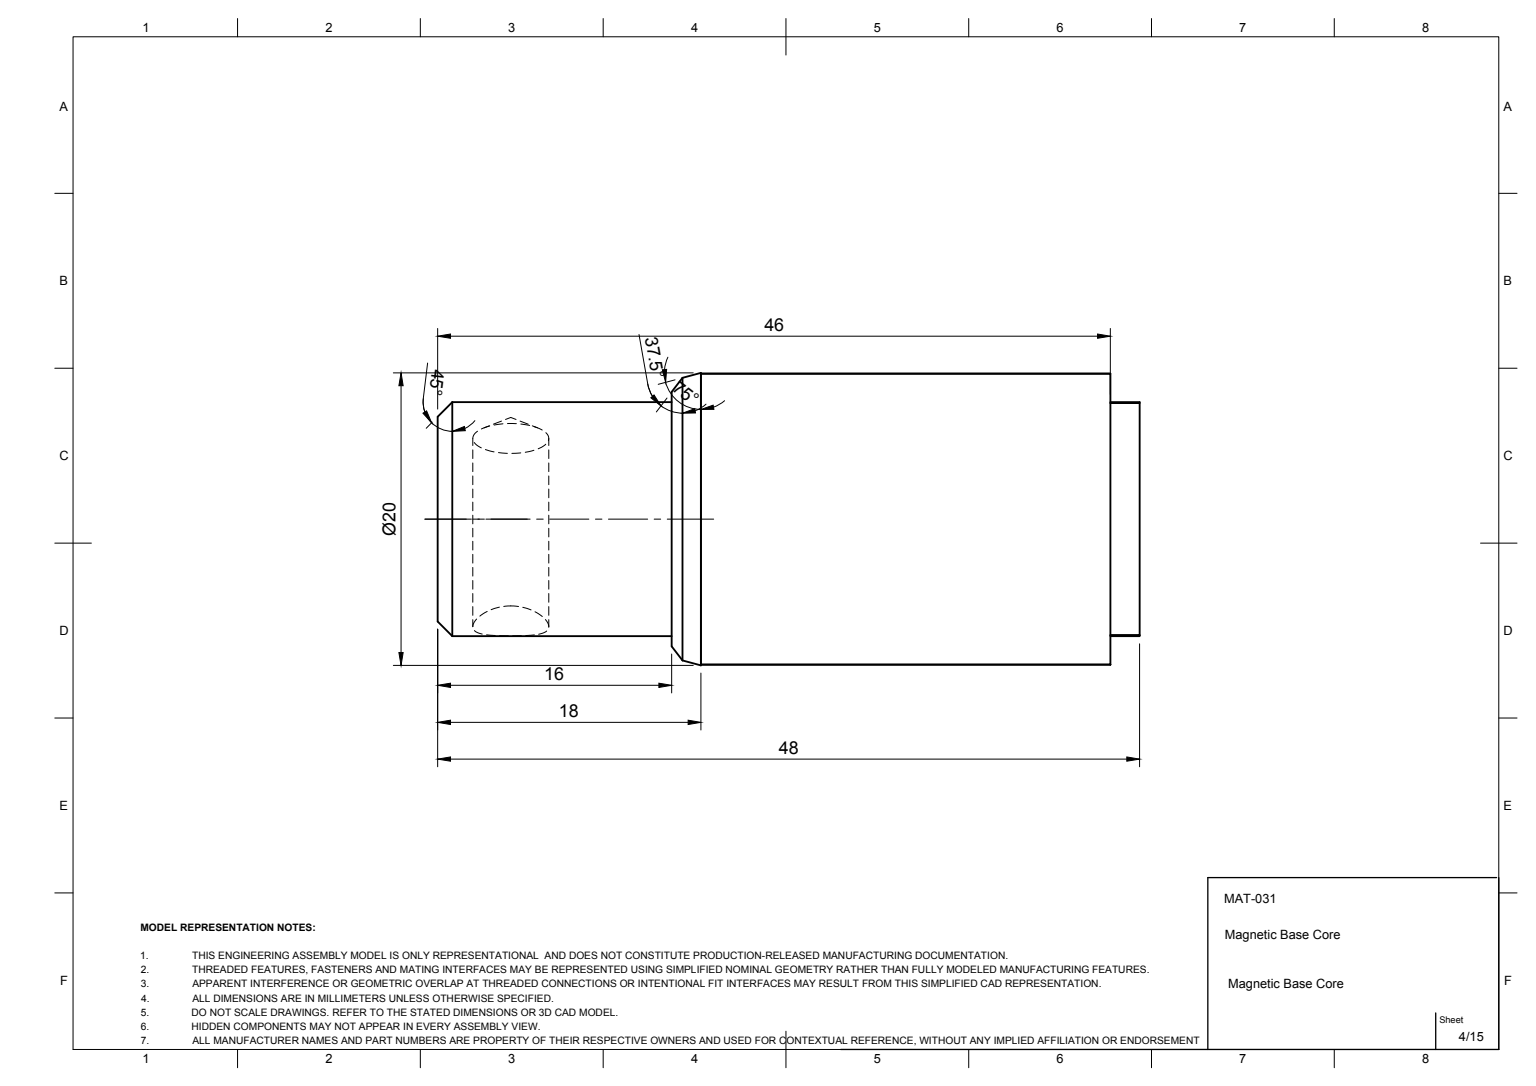
ISO-10303-21;
HEADER;
/* Generated by software containing ST-Developer
 * from STEP Tools, Inc. (www.steptools.com) 
 */

FILE_DESCRIPTION(
/* description */ ('STEP AP214'),
/* implementation_level */ '2;1');

FILE_NAME(
/* name */ 'Magnetic Base Core.step',
/* time_stamp */ '2026-11-14T06:58:01-08:00',
/* author */ (''),
/* organization */ (''),
/* preprocessor_version */ 'ST-DEVELOPER v20.2',
/* originating_system */ 'Autodesk Translation Framework v15.17.0.0',
/* authorisation */ '');

FILE_SCHEMA (('AUTOMOTIVE_DESIGN { 1 0 10303 214 3 1 1 }'));
ENDSEC;

DATA;
#10=MECHANICAL_DESIGN_GEOMETRIC_PRESENTATION_REPRESENTATION('',(#1144,#1145,#1146,#1147),#38635);
#862=FACE_BOUND('',#2714,.T.);
#863=FACE_BOUND('',#2717,.T.);
#907=B_SPLINE_CURVE_WITH_KNOTS('',3,(#24912,#24913,#24914,#24915,#24916,
#24917,#24918,#24919,#24920,#24921,#24922,#24923,#24924,#24925,#24926,#24927,
#24928,#24929,#24930,#24931,#24932,#24933,#24934,#24935,#24936,#24937,#24938,
#24939,#24940,#24941,#24942,#24943,#24944,#24945),.UNSPECIFIED.,.T.,.F.,
(4,2,2,2,2,2,2,2,2,2,2,2,2,2,2,2,4),(-1.57949026336004,-1.48075154424537,
-1.38201282513069,-1.28331526132536,-1.18461769752003,-1.08592013371471,
-0.98722256990938,-0.888483850794701,-0.789745131680022,-0.691006412565344,
-0.592267693450665,-0.493570129645338,-0.394872565840011,-0.296175002034684,
-0.197477438229357,-0.0987387191146787,0.),.UNSPECIFIED.);
#1018=CONICAL_SURFACE('',#17892,2.6,1.02974425867665);
#1019=CONICAL_SURFACE('',#17895,7.,0.785398163397448);
#1020=CONICAL_SURFACE('',#17898,8.69677462715879,0.916297857297022);
#1021=CONICAL_SURFACE('',#17904,10.,0.261799387799149);
#1113=SHAPE_REPRESENTATION_RELATIONSHIP('SRR','None',#38686,#1127);
#1127=ADVANCED_BREP_SHAPE_REPRESENTATION('',(#1170,#1171,#1172,#1173),#38622);
#1144=STYLED_ITEM('',(#38765),#1170);
#1145=STYLED_ITEM('',(#38765),#1171);
#1146=STYLED_ITEM('',(#38765),#1172);
#1147=STYLED_ITEM('',(#38765),#1173);
#1170=MANIFOLD_SOLID_BREP('Body1',#17610);
#1171=MANIFOLD_SOLID_BREP('Body2',#17611);
#1172=MANIFOLD_SOLID_BREP('Body3',#17612);
#1173=MANIFOLD_SOLID_BREP('Body4',#17613);
#1218=PLANE('',#17861);
#1219=PLANE('',#17863);
#1220=PLANE('',#17864);
#1221=PLANE('',#17865);
#1222=PLANE('',#17874);
#1223=PLANE('',#17875);
#1224=PLANE('',#17876);
#1225=PLANE('',#17877);
#1226=PLANE('',#17878);
#1227=PLANE('',#17879);
#1228=PLANE('',#17880);
#1229=PLANE('',#17881);
#1230=PLANE('',#17882);
#1231=PLANE('',#17885);
#1232=PLANE('',#17888);
#1233=PLANE('',#17889);
#1234=PLANE('',#17906);
#1235=PLANE('',#17907);
#1236=PLANE('',#17908);
#1681=FACE_OUTER_BOUND('',#2687,.T.);
#1682=FACE_OUTER_BOUND('',#2688,.T.);
#1683=FACE_OUTER_BOUND('',#2689,.T.);
#1684=FACE_OUTER_BOUND('',#2690,.T.);
#1685=FACE_OUTER_BOUND('',#2691,.T.);
#1686=FACE_OUTER_BOUND('',#2692,.T.);
#1687=FACE_OUTER_BOUND('',#2693,.T.);
#1688=FACE_OUTER_BOUND('',#2694,.T.);
#1689=FACE_OUTER_BOUND('',#2695,.T.);
#1690=FACE_OUTER_BOUND('',#2696,.T.);
#1691=FACE_OUTER_BOUND('',#2697,.T.);
#1692=FACE_OUTER_BOUND('',#2698,.T.);
#1693=FACE_OUTER_BOUND('',#2699,.T.);
#1694=FACE_OUTER_BOUND('',#2700,.T.);
#1695=FACE_OUTER_BOUND('',#2701,.T.);
#1696=FACE_OUTER_BOUND('',#2702,.T.);
#1697=FACE_OUTER_BOUND('',#2703,.T.);
#1698=FACE_OUTER_BOUND('',#2704,.T.);
#1699=FACE_OUTER_BOUND('',#2705,.T.);
#1700=FACE_OUTER_BOUND('',#2706,.T.);
#1701=FACE_OUTER_BOUND('',#2707,.T.);
#1702=FACE_OUTER_BOUND('',#2708,.T.);
#1703=FACE_OUTER_BOUND('',#2709,.T.);
#1704=FACE_OUTER_BOUND('',#2710,.T.);
#1705=FACE_OUTER_BOUND('',#2711,.T.);
#1706=FACE_OUTER_BOUND('',#2712,.T.);
#1707=FACE_OUTER_BOUND('',#2713,.T.);
#1708=FACE_OUTER_BOUND('',#2715,.T.);
#1709=FACE_OUTER_BOUND('',#2716,.T.);
#1710=FACE_OUTER_BOUND('',#2718,.T.);
#1711=FACE_OUTER_BOUND('',#2719,.T.);
#2687=EDGE_LOOP('',(#11101,#11102,#11103,#11104));
#2688=EDGE_LOOP('',(#11105,#11106));
#2689=EDGE_LOOP('',(#11107,#11108,#11109,#11110,#11111,#11112,#11113,#11114));
#2690=EDGE_LOOP('',(#11115,#11116));
#2691=EDGE_LOOP('',(#11117,#11118,#11119,#11120));
#2692=EDGE_LOOP('',(#11121,#11122,#11123,#11124));
#2693=EDGE_LOOP('',(#11125,#11126,#11127,#11128));
#2694=EDGE_LOOP('',(#11129,#11130,#11131,#11132));
#2695=EDGE_LOOP('',(#11133,#11134));
#2696=EDGE_LOOP('',(#11135,#11136,#11137,#11138,#11139,#11140,#11141,#11142));
#2697=EDGE_LOOP('',(#11143,#11144));
#2698=EDGE_LOOP('',(#11145,#11146,#11147,#11148));
#2699=EDGE_LOOP('',(#11149,#11150,#11151,#11152));
#2700=EDGE_LOOP('',(#11153,#11154,#11155,#11156,#11157,#11158,#11159,#11160));
#2701=EDGE_LOOP('',(#11161,#11162,#11163,#11164));
#2702=EDGE_LOOP('',(#11165,#11166,#11167,#11168,#11169,#11170,#11171,#11172));
#2703=EDGE_LOOP('',(#11173,#11174,#11175,#11176));
#2704=EDGE_LOOP('',(#11177,#11178,#11179,#11180));
#2705=EDGE_LOOP('',(#11181,#11182,#11183,#11184));
#2706=EDGE_LOOP('',(#11185,#11186,#11187,#11188));
#2707=EDGE_LOOP('',(#11189,#11190,#11191,#11192));
#2708=EDGE_LOOP('',(#11193,#11194,#11195,#11196));
#2709=EDGE_LOOP('',(#11197,#11198,#11199));
#2710=EDGE_LOOP('',(#11200,#11201,#11202,#11203));
#2711=EDGE_LOOP('',(#11204,#11205,#11206,#11207));
#2712=EDGE_LOOP('',(#11208,#11209,#11210,#11211,#11212));
#2713=EDGE_LOOP('',(#11213,#11214,#11215,#11216));
#2714=EDGE_LOOP('',(#11217));
#2715=EDGE_LOOP('',(#11218,#11219,#11220,#11221,#11222));
#2716=EDGE_LOOP('',(#11223));
#2717=EDGE_LOOP('',(#11224));
#2718=EDGE_LOOP('',(#11225));
#2719=EDGE_LOOP('',(#11226));
#3766=LINE('',#24807,#4710);
#3767=LINE('',#24810,#4711);
#3768=LINE('',#24815,#4712);
#3769=LINE('',#24818,#4713);
#3770=LINE('',#24819,#4714);
#3771=LINE('',#24821,#4715);
#3772=LINE('',#24822,#4716);
#3773=LINE('',#24823,#4717);
#3774=LINE('',#24833,#4718);
#3775=LINE('',#24836,#4719);
#3776=LINE('',#24842,#4720);
#3777=LINE('',#24845,#4721);
#3778=LINE('',#24847,#4722);
#3779=LINE('',#24849,#4723);
#3780=LINE('',#24850,#4724);
#3781=LINE('',#24851,#4725);
#3782=LINE('',#24857,#4726);
#3783=LINE('',#24859,#4727);
#3784=LINE('',#24861,#4728);
#3785=LINE('',#24862,#4729);
#3786=LINE('',#24866,#4730);
#3787=LINE('',#24868,#4731);
#3788=LINE('',#24870,#4732);
#3789=LINE('',#24872,#4733);
#3790=LINE('',#24874,#4734);
#3791=LINE('',#24875,#4735);
#3792=LINE('',#24876,#4736);
#3793=LINE('',#24880,#4737);
#3794=LINE('',#24881,#4738);
#3795=LINE('',#24882,#4739);
#3796=LINE('',#24885,#4740);
#3797=LINE('',#24887,#4741);
#3798=LINE('',#24889,#4742);
#3799=LINE('',#24891,#4743);
#3800=LINE('',#24892,#4744);
#3801=LINE('',#24893,#4745);
#3802=LINE('',#24907,#4746);
#3803=LINE('',#24911,#4747);
#3804=LINE('',#24950,#4748);
#3805=LINE('',#24958,#4749);
#3806=LINE('',#24963,#4750);
#3807=LINE('',#24967,#4751);
#4710=VECTOR('',#19957,1000.);
#4711=VECTOR('',#19960,1000.);
#4712=VECTOR('',#19965,1000.);
#4713=VECTOR('',#19968,1000.);
#4714=VECTOR('',#19969,1000.);
#4715=VECTOR('',#19970,1000.);
#4716=VECTOR('',#19971,1000.);
#4717=VECTOR('',#19972,1000.);
#4718=VECTOR('',#19985,1000.);
#4719=VECTOR('',#19988,1000.);
#4720=VECTOR('',#19993,1000.);
#4721=VECTOR('',#19996,1000.);
#4722=VECTOR('',#19999,1000.);
#4723=VECTOR('',#20002,1000.);
#4724=VECTOR('',#20003,1000.);
#4725=VECTOR('',#20004,1000.);
#4726=VECTOR('',#20011,1000.);
#4727=VECTOR('',#20012,1000.);
#4728=VECTOR('',#20013,1000.);
#4729=VECTOR('',#20014,1000.);
#4730=VECTOR('',#20017,1000.);
#4731=VECTOR('',#20018,1000.);
#4732=VECTOR('',#20019,1000.);
#4733=VECTOR('',#20020,1000.);
#4734=VECTOR('',#20021,1000.);
#4735=VECTOR('',#20022,1000.);
#4736=VECTOR('',#20023,1000.);
#4737=VECTOR('',#20026,1000.);
#4738=VECTOR('',#20027,1000.);
#4739=VECTOR('',#20028,1000.);
#4740=VECTOR('',#20031,1000.);
#4741=VECTOR('',#20032,1000.);
#4742=VECTOR('',#20033,1000.);
#4743=VECTOR('',#20034,1000.);
#4744=VECTOR('',#20035,1000.);
#4745=VECTOR('',#20036,1000.);
#4746=VECTOR('',#20059,2.6);
#4747=VECTOR('',#20064,2.6);
#4748=VECTOR('',#20069,7.);
#4749=VECTOR('',#20078,8.69677462715879);
#4750=VECTOR('',#20085,8.);
#4751=VECTOR('',#20090,10.);
#5614=CIRCLE('',#17859,10.);
#5615=CIRCLE('',#17860,10.);
#5616=CIRCLE('',#17862,8.);
#5617=CIRCLE('',#17866,8.);
#5618=CIRCLE('',#17869,8.);
#5619=CIRCLE('',#17870,8.);
#5620=CIRCLE('',#17872,10.);
#5621=CIRCLE('',#17873,10.);
#5622=CIRCLE('',#17883,8.);
#5623=CIRCLE('',#17884,8.);
#5624=CIRCLE('',#17887,8.);
#5625=CIRCLE('',#17890,8.);
#5626=CIRCLE('',#17893,2.6);
#5627=CIRCLE('',#17896,8.);
#5628=CIRCLE('',#17897,7.);
#5629=CIRCLE('',#17899,9.66270045344786);
#5630=CIRCLE('',#17900,9.66270045344786);
#5631=CIRCLE('',#17901,8.69677462715879);
#5632=CIRCLE('',#17903,8.);
#5633=CIRCLE('',#17905,10.);
#6576=VERTEX_POINT('',#24803);
#6577=VERTEX_POINT('',#24804);
#6578=VERTEX_POINT('',#24806);
#6579=VERTEX_POINT('',#24808);
#6580=VERTEX_POINT('',#24812);
#6581=VERTEX_POINT('',#24813);
#6582=VERTEX_POINT('',#24817);
#6583=VERTEX_POINT('',#24820);
#6584=VERTEX_POINT('',#24829);
#6585=VERTEX_POINT('',#24830);
#6586=VERTEX_POINT('',#24832);
#6587=VERTEX_POINT('',#24834);
#6588=VERTEX_POINT('',#24838);
#6589=VERTEX_POINT('',#24839);
#6590=VERTEX_POINT('',#24841);
#6591=VERTEX_POINT('',#24843);
#6592=VERTEX_POINT('',#24855);
#6593=VERTEX_POINT('',#24856);
#6594=VERTEX_POINT('',#24858);
#6595=VERTEX_POINT('',#24860);
#6596=VERTEX_POINT('',#24864);
#6597=VERTEX_POINT('',#24865);
#6598=VERTEX_POINT('',#24867);
#6599=VERTEX_POINT('',#24869);
#6600=VERTEX_POINT('',#24871);
#6601=VERTEX_POINT('',#24873);
#6602=VERTEX_POINT('',#24878);
#6603=VERTEX_POINT('',#24879);
#6604=VERTEX_POINT('',#24884);
#6605=VERTEX_POINT('',#24886);
#6606=VERTEX_POINT('',#24888);
#6607=VERTEX_POINT('',#24890);
#6608=VERTEX_POINT('',#24905);
#6609=VERTEX_POINT('',#24906);
#6610=VERTEX_POINT('',#24910);
#6611=VERTEX_POINT('',#24947);
#6612=VERTEX_POINT('',#24949);
#6613=VERTEX_POINT('',#24953);
#6614=VERTEX_POINT('',#24954);
#6615=VERTEX_POINT('',#24957);
#6616=VERTEX_POINT('',#24961);
#6617=VERTEX_POINT('',#24965);
#8337=EDGE_CURVE('',#6576,#6577,#5614,.T.);
#8338=EDGE_CURVE('',#6576,#6578,#3766,.T.);
#8339=EDGE_CURVE('',#6579,#6578,#5615,.T.);
#8340=EDGE_CURVE('',#6579,#6577,#3767,.T.);
#8341=EDGE_CURVE('',#6580,#6581,#5616,.T.);
#8342=EDGE_CURVE('',#6581,#6580,#3768,.T.);
#8343=EDGE_CURVE('',#6577,#6582,#3769,.T.);
#8344=EDGE_CURVE('',#6579,#6578,#3770,.T.);
#8345=EDGE_CURVE('',#6583,#6576,#3771,.T.);
#8346=EDGE_CURVE('',#6580,#6583,#3772,.T.);
#8347=EDGE_CURVE('',#6582,#6581,#3773,.T.);
#8348=EDGE_CURVE('',#6583,#6582,#5617,.T.);
#8349=EDGE_CURVE('',#6584,#6585,#5618,.T.);
#8350=EDGE_CURVE('',#6585,#6586,#3774,.T.);
#8351=EDGE_CURVE('',#6587,#6586,#5619,.T.);
#8352=EDGE_CURVE('',#6587,#6584,#3775,.T.);
#8353=EDGE_CURVE('',#6588,#6589,#5620,.T.);
#8354=EDGE_CURVE('',#6588,#6590,#3776,.T.);
#8355=EDGE_CURVE('',#6591,#6590,#5621,.T.);
#8356=EDGE_CURVE('',#6591,#6589,#3777,.T.);
#8357=EDGE_CURVE('',#6586,#6587,#3778,.T.);
#8358=EDGE_CURVE('',#6590,#6585,#3779,.T.);
#8359=EDGE_CURVE('',#6588,#6589,#3780,.T.);
#8360=EDGE_CURVE('',#6584,#6591,#3781,.T.);
#8361=EDGE_CURVE('',#6592,#6593,#3782,.T.);
#8362=EDGE_CURVE('',#6592,#6594,#3783,.T.);
#8363=EDGE_CURVE('',#6594,#6595,#3784,.T.);
#8364=EDGE_CURVE('',#6593,#6595,#3785,.T.);
#8365=EDGE_CURVE('',#6596,#6597,#3786,.T.);
#8366=EDGE_CURVE('',#6596,#6598,#3787,.T.);
#8367=EDGE_CURVE('',#6598,#6599,#3788,.T.);
#8368=EDGE_CURVE('',#6599,#6600,#3789,.T.);
#8369=EDGE_CURVE('',#6600,#6601,#3790,.T.);
#8370=EDGE_CURVE('',#6601,#6592,#3791,.T.);
#8371=EDGE_CURVE('',#6597,#6593,#3792,.T.);
#8372=EDGE_CURVE('',#6602,#6603,#3793,.T.);
#8373=EDGE_CURVE('',#6602,#6596,#3794,.T.);
#8374=EDGE_CURVE('',#6603,#6597,#3795,.T.);
#8375=EDGE_CURVE('',#6594,#6604,#3796,.T.);
#8376=EDGE_CURVE('',#6604,#6605,#3797,.T.);
#8377=EDGE_CURVE('',#6605,#6606,#3798,.T.);
#8378=EDGE_CURVE('',#6606,#6607,#3799,.T.);
#8379=EDGE_CURVE('',#6607,#6602,#3800,.T.);
#8380=EDGE_CURVE('',#6595,#6603,#3801,.T.);
#8381=EDGE_CURVE('',#6605,#6600,#5622,.T.);
#8382=EDGE_CURVE('',#6599,#6606,#5623,.T.);
#8383=EDGE_CURVE('',#6598,#6607,#5624,.T.);
#8384=EDGE_CURVE('',#6604,#6601,#5625,.T.);
#8385=EDGE_CURVE('',#6608,#6609,#3802,.T.);
#8386=EDGE_CURVE('',#6609,#6609,#5626,.T.);
#8387=EDGE_CURVE('',#6609,#6610,#3803,.T.);
#8388=EDGE_CURVE('',#6610,#6610,#907,.T.);
#8389=EDGE_CURVE('',#6611,#6611,#5627,.T.);
#8390=EDGE_CURVE('',#6611,#6612,#3804,.T.);
#8391=EDGE_CURVE('',#6612,#6612,#5628,.T.);
#8392=EDGE_CURVE('',#6613,#6614,#5629,.T.);
#8393=EDGE_CURVE('',#6614,#6613,#5630,.T.);
#8394=EDGE_CURVE('',#6614,#6615,#3805,.T.);
#8395=EDGE_CURVE('',#6615,#6615,#5631,.T.);
#8396=EDGE_CURVE('',#6616,#6616,#5632,.T.);
#8397=EDGE_CURVE('',#6616,#6611,#3806,.T.);
#8398=EDGE_CURVE('',#6617,#6617,#5633,.T.);
#8399=EDGE_CURVE('',#6617,#6613,#3807,.T.);
#11101=ORIENTED_EDGE('',*,*,#8337,.F.);
#11102=ORIENTED_EDGE('',*,*,#8338,.T.);
#11103=ORIENTED_EDGE('',*,*,#8339,.F.);
#11104=ORIENTED_EDGE('',*,*,#8340,.T.);
#11105=ORIENTED_EDGE('',*,*,#8341,.T.);
#11106=ORIENTED_EDGE('',*,*,#8342,.T.);
#11107=ORIENTED_EDGE('',*,*,#8343,.F.);
#11108=ORIENTED_EDGE('',*,*,#8340,.F.);
#11109=ORIENTED_EDGE('',*,*,#8344,.T.);
#11110=ORIENTED_EDGE('',*,*,#8338,.F.);
#11111=ORIENTED_EDGE('',*,*,#8345,.F.);
#11112=ORIENTED_EDGE('',*,*,#8346,.F.);
#11113=ORIENTED_EDGE('',*,*,#8342,.F.);
#11114=ORIENTED_EDGE('',*,*,#8347,.F.);
#11115=ORIENTED_EDGE('',*,*,#8344,.F.);
#11116=ORIENTED_EDGE('',*,*,#8339,.T.);
#11117=ORIENTED_EDGE('',*,*,#8343,.T.);
#11118=ORIENTED_EDGE('',*,*,#8348,.F.);
#11119=ORIENTED_EDGE('',*,*,#8345,.T.);
#11120=ORIENTED_EDGE('',*,*,#8337,.T.);
#11121=ORIENTED_EDGE('',*,*,#8347,.T.);
#11122=ORIENTED_EDGE('',*,*,#8341,.F.);
#11123=ORIENTED_EDGE('',*,*,#8346,.T.);
#11124=ORIENTED_EDGE('',*,*,#8348,.T.);
#11125=ORIENTED_EDGE('',*,*,#8349,.T.);
#11126=ORIENTED_EDGE('',*,*,#8350,.T.);
#11127=ORIENTED_EDGE('',*,*,#8351,.F.);
#11128=ORIENTED_EDGE('',*,*,#8352,.T.);
#11129=ORIENTED_EDGE('',*,*,#8353,.F.);
#11130=ORIENTED_EDGE('',*,*,#8354,.T.);
#11131=ORIENTED_EDGE('',*,*,#8355,.F.);
#11132=ORIENTED_EDGE('',*,*,#8356,.T.);
#11133=ORIENTED_EDGE('',*,*,#8351,.T.);
#11134=ORIENTED_EDGE('',*,*,#8357,.T.);
#11135=ORIENTED_EDGE('',*,*,#8358,.F.);
#11136=ORIENTED_EDGE('',*,*,#8354,.F.);
#11137=ORIENTED_EDGE('',*,*,#8359,.T.);
#11138=ORIENTED_EDGE('',*,*,#8356,.F.);
#11139=ORIENTED_EDGE('',*,*,#8360,.F.);
#11140=ORIENTED_EDGE('',*,*,#8352,.F.);
#11141=ORIENTED_EDGE('',*,*,#8357,.F.);
#11142=ORIENTED_EDGE('',*,*,#8350,.F.);
#11143=ORIENTED_EDGE('',*,*,#8359,.F.);
#11144=ORIENTED_EDGE('',*,*,#8353,.T.);
#11145=ORIENTED_EDGE('',*,*,#8358,.T.);
#11146=ORIENTED_EDGE('',*,*,#8349,.F.);
#11147=ORIENTED_EDGE('',*,*,#8360,.T.);
#11148=ORIENTED_EDGE('',*,*,#8355,.T.);
#11149=ORIENTED_EDGE('',*,*,#8361,.F.);
#11150=ORIENTED_EDGE('',*,*,#8362,.T.);
#11151=ORIENTED_EDGE('',*,*,#8363,.T.);
#11152=ORIENTED_EDGE('',*,*,#8364,.F.);
#11153=ORIENTED_EDGE('',*,*,#8365,.F.);
#11154=ORIENTED_EDGE('',*,*,#8366,.T.);
#11155=ORIENTED_EDGE('',*,*,#8367,.T.);
#11156=ORIENTED_EDGE('',*,*,#8368,.T.);
#11157=ORIENTED_EDGE('',*,*,#8369,.T.);
#11158=ORIENTED_EDGE('',*,*,#8370,.T.);
#11159=ORIENTED_EDGE('',*,*,#8361,.T.);
#11160=ORIENTED_EDGE('',*,*,#8371,.F.);
#11161=ORIENTED_EDGE('',*,*,#8372,.F.);
#11162=ORIENTED_EDGE('',*,*,#8373,.T.);
#11163=ORIENTED_EDGE('',*,*,#8365,.T.);
#11164=ORIENTED_EDGE('',*,*,#8374,.F.);
#11165=ORIENTED_EDGE('',*,*,#8363,.F.);
#11166=ORIENTED_EDGE('',*,*,#8375,.T.);
#11167=ORIENTED_EDGE('',*,*,#8376,.T.);
#11168=ORIENTED_EDGE('',*,*,#8377,.T.);
#11169=ORIENTED_EDGE('',*,*,#8378,.T.);
#11170=ORIENTED_EDGE('',*,*,#8379,.T.);
#11171=ORIENTED_EDGE('',*,*,#8372,.T.);
#11172=ORIENTED_EDGE('',*,*,#8380,.F.);
#11173=ORIENTED_EDGE('',*,*,#8377,.F.);
#11174=ORIENTED_EDGE('',*,*,#8381,.T.);
#11175=ORIENTED_EDGE('',*,*,#8368,.F.);
#11176=ORIENTED_EDGE('',*,*,#8382,.T.);
#11177=ORIENTED_EDGE('',*,*,#8364,.T.);
#11178=ORIENTED_EDGE('',*,*,#8380,.T.);
#11179=ORIENTED_EDGE('',*,*,#8374,.T.);
#11180=ORIENTED_EDGE('',*,*,#8371,.T.);
#11181=ORIENTED_EDGE('',*,*,#8383,.T.);
#11182=ORIENTED_EDGE('',*,*,#8378,.F.);
#11183=ORIENTED_EDGE('',*,*,#8382,.F.);
#11184=ORIENTED_EDGE('',*,*,#8367,.F.);
#11185=ORIENTED_EDGE('',*,*,#8373,.F.);
#11186=ORIENTED_EDGE('',*,*,#8379,.F.);
#11187=ORIENTED_EDGE('',*,*,#8383,.F.);
#11188=ORIENTED_EDGE('',*,*,#8366,.F.);
#11189=ORIENTED_EDGE('',*,*,#8384,.F.);
#11190=ORIENTED_EDGE('',*,*,#8375,.F.);
#11191=ORIENTED_EDGE('',*,*,#8362,.F.);
#11192=ORIENTED_EDGE('',*,*,#8370,.F.);
#11193=ORIENTED_EDGE('',*,*,#8381,.F.);
#11194=ORIENTED_EDGE('',*,*,#8376,.F.);
#11195=ORIENTED_EDGE('',*,*,#8384,.T.);
#11196=ORIENTED_EDGE('',*,*,#8369,.F.);
#11197=ORIENTED_EDGE('',*,*,#8385,.T.);
#11198=ORIENTED_EDGE('',*,*,#8386,.T.);
#11199=ORIENTED_EDGE('',*,*,#8385,.F.);
#11200=ORIENTED_EDGE('',*,*,#8386,.F.);
#11201=ORIENTED_EDGE('',*,*,#8387,.T.);
#11202=ORIENTED_EDGE('',*,*,#8388,.F.);
#11203=ORIENTED_EDGE('',*,*,#8387,.F.);
#11204=ORIENTED_EDGE('',*,*,#8389,.F.);
#11205=ORIENTED_EDGE('',*,*,#8390,.T.);
#11206=ORIENTED_EDGE('',*,*,#8391,.F.);
#11207=ORIENTED_EDGE('',*,*,#8390,.F.);
#11208=ORIENTED_EDGE('',*,*,#8392,.F.);
#11209=ORIENTED_EDGE('',*,*,#8393,.F.);
#11210=ORIENTED_EDGE('',*,*,#8394,.T.);
#11211=ORIENTED_EDGE('',*,*,#8395,.F.);
#11212=ORIENTED_EDGE('',*,*,#8394,.F.);
#11213=ORIENTED_EDGE('',*,*,#8396,.T.);
#11214=ORIENTED_EDGE('',*,*,#8397,.T.);
#11215=ORIENTED_EDGE('',*,*,#8389,.T.);
#11216=ORIENTED_EDGE('',*,*,#8397,.F.);
#11217=ORIENTED_EDGE('',*,*,#8388,.T.);
#11218=ORIENTED_EDGE('',*,*,#8398,.T.);
#11219=ORIENTED_EDGE('',*,*,#8399,.T.);
#11220=ORIENTED_EDGE('',*,*,#8392,.T.);
#11221=ORIENTED_EDGE('',*,*,#8393,.T.);
#11222=ORIENTED_EDGE('',*,*,#8399,.F.);
#11223=ORIENTED_EDGE('',*,*,#8395,.T.);
#11224=ORIENTED_EDGE('',*,*,#8396,.F.);
#11225=ORIENTED_EDGE('',*,*,#8398,.F.);
#11226=ORIENTED_EDGE('',*,*,#8391,.T.);
#16259=CYLINDRICAL_SURFACE('',#17858,10.);
#16260=CYLINDRICAL_SURFACE('',#17867,8.);
#16261=CYLINDRICAL_SURFACE('',#17868,8.);
#16262=CYLINDRICAL_SURFACE('',#17871,10.);
#16263=CYLINDRICAL_SURFACE('',#17886,8.);
#16264=CYLINDRICAL_SURFACE('',#17891,8.);
#16265=CYLINDRICAL_SURFACE('',#17894,2.6);
#16266=CYLINDRICAL_SURFACE('',#17902,8.);
#16640=ADVANCED_FACE('',(#1681),#16259,.T.);
#16641=ADVANCED_FACE('',(#1682),#1218,.F.);
#16642=ADVANCED_FACE('',(#1683),#1219,.F.);
#16643=ADVANCED_FACE('',(#1684),#1220,.T.);
#16644=ADVANCED_FACE('',(#1685),#1221,.T.);
#16645=ADVANCED_FACE('',(#1686),#16260,.T.);
#16646=ADVANCED_FACE('',(#1687),#16261,.T.);
#16647=ADVANCED_FACE('',(#1688),#16262,.T.);
#16648=ADVANCED_FACE('',(#1689),#1222,.F.);
#16649=ADVANCED_FACE('',(#1690),#1223,.F.);
#16650=ADVANCED_FACE('',(#1691),#1224,.T.);
#16651=ADVANCED_FACE('',(#1692),#1225,.T.);
#16652=ADVANCED_FACE('',(#1693),#1226,.T.);
#16653=ADVANCED_FACE('',(#1694),#1227,.T.);
#16654=ADVANCED_FACE('',(#1695),#1228,.T.);
#16655=ADVANCED_FACE('',(#1696),#1229,.T.);
#16656=ADVANCED_FACE('',(#1697),#1230,.T.);
#16657=ADVANCED_FACE('',(#1698),#1231,.F.);
#16658=ADVANCED_FACE('',(#1699),#16263,.T.);
#16659=ADVANCED_FACE('',(#1700),#1232,.T.);
#16660=ADVANCED_FACE('',(#1701),#1233,.T.);
#16661=ADVANCED_FACE('',(#1702),#16264,.T.);
#16662=ADVANCED_FACE('',(#1703),#1018,.F.);
#16663=ADVANCED_FACE('',(#1704),#16265,.F.);
#16664=ADVANCED_FACE('',(#1705),#1019,.T.);
#16665=ADVANCED_FACE('',(#1706),#1020,.T.);
#16666=ADVANCED_FACE('',(#1707,#862),#16266,.T.);
#16667=ADVANCED_FACE('',(#1708),#1021,.T.);
#16668=ADVANCED_FACE('',(#1709,#863),#1234,.T.);
#16669=ADVANCED_FACE('',(#1710),#1235,.F.);
#16670=ADVANCED_FACE('',(#1711),#1236,.T.);
#17610=CLOSED_SHELL('',(#16640,#16641,#16642,#16643,#16644,#16645));
#17611=CLOSED_SHELL('',(#16646,#16647,#16648,#16649,#16650,#16651));
#17612=CLOSED_SHELL('',(#16652,#16653,#16654,#16655,#16656,#16657,#16658,
#16659,#16660,#16661));
#17613=CLOSED_SHELL('',(#16662,#16663,#16664,#16665,#16666,#16667,#16668,
#16669,#16670));
#17857=AXIS2_PLACEMENT_3D('',#24801,#19951,#19952);
#17858=AXIS2_PLACEMENT_3D('',#24802,#19953,#19954);
#17859=AXIS2_PLACEMENT_3D('',#24805,#19955,#19956);
#17860=AXIS2_PLACEMENT_3D('',#24809,#19958,#19959);
#17861=AXIS2_PLACEMENT_3D('',#24811,#19961,#19962);
#17862=AXIS2_PLACEMENT_3D('',#24814,#19963,#19964);
#17863=AXIS2_PLACEMENT_3D('',#24816,#19966,#19967);
#17864=AXIS2_PLACEMENT_3D('',#24824,#19973,#19974);
#17865=AXIS2_PLACEMENT_3D('',#24825,#19975,#19976);
#17866=AXIS2_PLACEMENT_3D('',#24826,#19977,#19978);
#17867=AXIS2_PLACEMENT_3D('',#24827,#19979,#19980);
#17868=AXIS2_PLACEMENT_3D('',#24828,#19981,#19982);
#17869=AXIS2_PLACEMENT_3D('',#24831,#19983,#19984);
#17870=AXIS2_PLACEMENT_3D('',#24835,#19986,#19987);
#17871=AXIS2_PLACEMENT_3D('',#24837,#19989,#19990);
#17872=AXIS2_PLACEMENT_3D('',#24840,#19991,#19992);
#17873=AXIS2_PLACEMENT_3D('',#24844,#19994,#19995);
#17874=AXIS2_PLACEMENT_3D('',#24846,#19997,#19998);
#17875=AXIS2_PLACEMENT_3D('',#24848,#20000,#20001);
#17876=AXIS2_PLACEMENT_3D('',#24852,#20005,#20006);
#17877=AXIS2_PLACEMENT_3D('',#24853,#20007,#20008);
#17878=AXIS2_PLACEMENT_3D('',#24854,#20009,#20010);
#17879=AXIS2_PLACEMENT_3D('',#24863,#20015,#20016);
#17880=AXIS2_PLACEMENT_3D('',#24877,#20024,#20025);
#17881=AXIS2_PLACEMENT_3D('',#24883,#20029,#20030);
#17882=AXIS2_PLACEMENT_3D('',#24894,#20037,#20038);
#17883=AXIS2_PLACEMENT_3D('',#24895,#20039,#20040);
#17884=AXIS2_PLACEMENT_3D('',#24896,#20041,#20042);
#17885=AXIS2_PLACEMENT_3D('',#24897,#20043,#20044);
#17886=AXIS2_PLACEMENT_3D('',#24898,#20045,#20046);
#17887=AXIS2_PLACEMENT_3D('',#24899,#20047,#20048);
#17888=AXIS2_PLACEMENT_3D('',#24900,#20049,#20050);
#17889=AXIS2_PLACEMENT_3D('',#24901,#20051,#20052);
#17890=AXIS2_PLACEMENT_3D('',#24902,#20053,#20054);
#17891=AXIS2_PLACEMENT_3D('',#24903,#20055,#20056);
#17892=AXIS2_PLACEMENT_3D('',#24904,#20057,#20058);
#17893=AXIS2_PLACEMENT_3D('',#24908,#20060,#20061);
#17894=AXIS2_PLACEMENT_3D('',#24909,#20062,#20063);
#17895=AXIS2_PLACEMENT_3D('',#24946,#20065,#20066);
#17896=AXIS2_PLACEMENT_3D('',#24948,#20067,#20068);
#17897=AXIS2_PLACEMENT_3D('',#24951,#20070,#20071);
#17898=AXIS2_PLACEMENT_3D('',#24952,#20072,#20073);
#17899=AXIS2_PLACEMENT_3D('',#24955,#20074,#20075);
#17900=AXIS2_PLACEMENT_3D('',#24956,#20076,#20077);
#17901=AXIS2_PLACEMENT_3D('',#24959,#20079,#20080);
#17902=AXIS2_PLACEMENT_3D('',#24960,#20081,#20082);
#17903=AXIS2_PLACEMENT_3D('',#24962,#20083,#20084);
#17904=AXIS2_PLACEMENT_3D('',#24964,#20086,#20087);
#17905=AXIS2_PLACEMENT_3D('',#24966,#20088,#20089);
#17906=AXIS2_PLACEMENT_3D('',#24968,#20091,#20092);
#17907=AXIS2_PLACEMENT_3D('',#24969,#20093,#20094);
#17908=AXIS2_PLACEMENT_3D('',#24970,#20095,#20096);
#19951=DIRECTION('axis',(0.,0.,1.));
#19952=DIRECTION('refdir',(1.,0.,0.));
#19953=DIRECTION('center_axis',(0.,-1.,0.));
#19954=DIRECTION('ref_axis',(1.22464679914735E-16,0.,1.));
#19955=DIRECTION('center_axis',(0.,-1.,0.));
#19956=DIRECTION('ref_axis',(0.,0.,-1.));
#19957=DIRECTION('',(0.,1.,0.));
#19958=DIRECTION('center_axis',(0.,1.,0.));
#19959=DIRECTION('ref_axis',(0.,0.,1.));
#19960=DIRECTION('',(0.,-1.,0.));
#19961=DIRECTION('center_axis',(0.,1.,0.));
#19962=DIRECTION('ref_axis',(0.,0.,1.));
#19963=DIRECTION('center_axis',(0.,-1.,0.));
#19964=DIRECTION('ref_axis',(0.,0.,-1.));
#19965=DIRECTION('',(1.,0.,0.));
#19966=DIRECTION('center_axis',(0.,0.,1.));
#19967=DIRECTION('ref_axis',(1.,0.,0.));
#19968=DIRECTION('',(1.,0.,0.));
#19969=DIRECTION('',(1.,0.,0.));
#19970=DIRECTION('',(1.,0.,0.));
#19971=DIRECTION('',(0.,1.,0.));
#19972=DIRECTION('',(0.,-1.,0.));
#19973=DIRECTION('center_axis',(0.,1.,0.));
#19974=DIRECTION('ref_axis',(0.,0.,1.));
#19975=DIRECTION('center_axis',(0.,-1.,0.));
#19976=DIRECTION('ref_axis',(0.,0.,-1.));
#19977=DIRECTION('center_axis',(0.,-1.,0.));
#19978=DIRECTION('ref_axis',(0.,0.,-1.));
#19979=DIRECTION('center_axis',(0.,-1.,0.));
#19980=DIRECTION('ref_axis',(-1.22464679914735E-16,0.,1.));
#19981=DIRECTION('center_axis',(0.,-1.,0.));
#19982=DIRECTION('ref_axis',(0.,0.,-1.));
#19983=DIRECTION('center_axis',(0.,-1.,0.));
#19984=DIRECTION('ref_axis',(0.,0.,-1.));
#19985=DIRECTION('',(0.,-1.,0.));
#19986=DIRECTION('center_axis',(0.,-1.,0.));
#19987=DIRECTION('ref_axis',(0.,0.,-1.));
#19988=DIRECTION('',(0.,1.,0.));
#19989=DIRECTION('center_axis',(0.,-1.,0.));
#19990=DIRECTION('ref_axis',(0.,0.,-1.));
#19991=DIRECTION('center_axis',(0.,1.,0.));
#19992=DIRECTION('ref_axis',(0.,0.,1.));
#19993=DIRECTION('',(0.,-1.,0.));
#19994=DIRECTION('center_axis',(0.,-1.,0.));
#19995=DIRECTION('ref_axis',(0.,0.,-1.));
#19996=DIRECTION('',(0.,1.,0.));
#19997=DIRECTION('center_axis',(0.,1.,0.));
#19998=DIRECTION('ref_axis',(0.,0.,1.));
#19999=DIRECTION('',(-1.,0.,0.));
#20000=DIRECTION('center_axis',(0.,0.,-1.));
#20001=DIRECTION('ref_axis',(-1.,0.,0.));
#20002=DIRECTION('',(-1.,0.,0.));
#20003=DIRECTION('',(-1.,0.,0.));
#20004=DIRECTION('',(-1.,0.,0.));
#20005=DIRECTION('center_axis',(0.,1.,0.));
#20006=DIRECTION('ref_axis',(0.,0.,1.));
#20007=DIRECTION('center_axis',(0.,-1.,0.));
#20008=DIRECTION('ref_axis',(0.,0.,-1.));
#20009=DIRECTION('center_axis',(1.,0.,0.));
#20010=DIRECTION('ref_axis',(0.,0.,-1.));
#20011=DIRECTION('',(0.,1.,0.));
#20012=DIRECTION('',(0.,0.,-1.));
#20013=DIRECTION('',(0.,1.,0.));
#20014=DIRECTION('',(0.,0.,-1.));
#20015=DIRECTION('center_axis',(0.,0.,1.));
#20016=DIRECTION('ref_axis',(1.,0.,0.));
#20017=DIRECTION('',(0.,1.,0.));
#20018=DIRECTION('',(1.,0.,0.));
#20019=DIRECTION('',(0.,-1.,0.));
#20020=DIRECTION('',(1.,0.,0.));
#20021=DIRECTION('',(0.,1.,0.));
#20022=DIRECTION('',(1.,0.,0.));
#20023=DIRECTION('',(1.,0.,0.));
#20024=DIRECTION('center_axis',(-1.,0.,0.));
#20025=DIRECTION('ref_axis',(0.,0.,1.));
#20026=DIRECTION('',(0.,1.,0.));
#20027=DIRECTION('',(0.,0.,1.));
#20028=DIRECTION('',(0.,0.,1.));
#20029=DIRECTION('center_axis',(0.,0.,-1.));
#20030=DIRECTION('ref_axis',(-1.,0.,0.));
#20031=DIRECTION('',(-1.,0.,0.));
#20032=DIRECTION('',(0.,-1.,0.));
#20033=DIRECTION('',(-1.,0.,0.));
#20034=DIRECTION('',(0.,1.,0.));
#20035=DIRECTION('',(-1.,0.,0.));
#20036=DIRECTION('',(-1.,0.,0.));
#20037=DIRECTION('center_axis',(0.,-1.,0.));
#20038=DIRECTION('ref_axis',(0.,0.,-1.));
#20039=DIRECTION('center_axis',(0.,-1.,0.));
#20040=DIRECTION('ref_axis',(0.,0.,-1.));
#20041=DIRECTION('center_axis',(0.,-1.,0.));
#20042=DIRECTION('ref_axis',(0.,0.,-1.));
#20043=DIRECTION('center_axis',(0.,-1.,0.));
#20044=DIRECTION('ref_axis',(0.,0.,-1.));
#20045=DIRECTION('center_axis',(0.,-1.,0.));
#20046=DIRECTION('ref_axis',(0.,0.,-1.));
#20047=DIRECTION('center_axis',(0.,-1.,0.));
#20048=DIRECTION('ref_axis',(0.,0.,-1.));
#20049=DIRECTION('center_axis',(0.,-1.,0.));
#20050=DIRECTION('ref_axis',(0.,0.,-1.));
#20051=DIRECTION('center_axis',(0.,-1.,0.));
#20052=DIRECTION('ref_axis',(0.,0.,-1.));
#20053=DIRECTION('center_axis',(0.,-1.,0.));
#20054=DIRECTION('ref_axis',(0.,0.,-1.));
#20055=DIRECTION('center_axis',(0.,-1.,0.));
#20056=DIRECTION('ref_axis',(0.,0.,-1.));
#20057=DIRECTION('center_axis',(-0.91945378174003,0.,-0.39319809669422));
#20058=DIRECTION('ref_axis',(-0.39319809669422,0.,0.91945378174003));
#20059=DIRECTION('',(-0.136517154531564,-1.04972719113862E-16,-0.990637706994139));
#20060=DIRECTION('center_axis',(-0.91945378174003,0.,-0.39319809669422));
#20061=DIRECTION('ref_axis',(-0.39319809669422,0.,0.91945378174003));
#20062=DIRECTION('center_axis',(-0.91945378174003,0.,-0.39319809669422));
#20063=DIRECTION('ref_axis',(-0.39319809669422,0.,0.91945378174003));
#20064=DIRECTION('',(-0.91945378174003,0.,-0.39319809669422));
#20065=DIRECTION('center_axis',(0.,-1.,0.));
#20066=DIRECTION('ref_axis',(0.,0.,-1.));
#20067=DIRECTION('center_axis',(0.,-1.,0.));
#20068=DIRECTION('ref_axis',(0.,0.,1.));
#20069=DIRECTION('',(8.65956056235493E-17,0.707106781186548,-0.707106781186547));
#20070=DIRECTION('center_axis',(0.,1.,0.));
#20071=DIRECTION('ref_axis',(0.,0.,1.));
#20072=DIRECTION('center_axis',(0.,-1.,0.));
#20073=DIRECTION('ref_axis',(0.,0.,-1.));
#20074=DIRECTION('center_axis',(0.,-1.,0.));
#20075=DIRECTION('ref_axis',(0.,0.,-1.));
#20076=DIRECTION('center_axis',(0.,-1.,0.));
#20077=DIRECTION('ref_axis',(0.,0.,-1.));
#20078=DIRECTION('',(9.71577628780521E-17,0.608761429008721,-0.793353340291235));
#20079=DIRECTION('center_axis',(0.,1.,0.));
#20080=DIRECTION('ref_axis',(0.,0.,1.));
#20081=DIRECTION('center_axis',(0.,-1.,0.));
#20082=DIRECTION('ref_axis',(0.,0.,-1.));
#20083=DIRECTION('center_axis',(0.,1.,0.));
#20084=DIRECTION('ref_axis',(0.,0.,1.));
#20085=DIRECTION('',(0.,1.,0.));
#20086=DIRECTION('center_axis',(0.,-1.,0.));
#20087=DIRECTION('ref_axis',(0.,0.,1.));
#20088=DIRECTION('center_axis',(0.,1.,0.));
#20089=DIRECTION('ref_axis',(0.,0.,1.));
#20090=DIRECTION('',(-3.16961915143177E-17,0.965925826289068,0.258819045102521));
#20091=DIRECTION('center_axis',(0.,1.,0.));
#20092=DIRECTION('ref_axis',(0.,0.,1.));
#20093=DIRECTION('center_axis',(0.,1.,0.));
#20094=DIRECTION('ref_axis',(0.,0.,1.));
#20095=DIRECTION('center_axis',(0.,1.,0.));
#20096=DIRECTION('ref_axis',(0.,0.,1.));
#24801=CARTESIAN_POINT('',(0.,0.,0.));
#24802=CARTESIAN_POINT('Origin',(0.,30.,0.));
#24803=CARTESIAN_POINT('',(9.9498743710662,2.,1.));
#24804=CARTESIAN_POINT('',(-9.9498743710662,2.,1.));
#24805=CARTESIAN_POINT('Origin',(0.,2.,0.));
#24806=CARTESIAN_POINT('',(9.94987437106619,30.,1.));
#24807=CARTESIAN_POINT('',(9.9498743710662,30.,1.));
#24808=CARTESIAN_POINT('',(-9.9498743710662,30.,1.));
#24809=CARTESIAN_POINT('Origin',(0.,30.,0.));
#24810=CARTESIAN_POINT('',(-9.9498743710662,30.,1.));
#24811=CARTESIAN_POINT('Origin',(0.,0.,0.));
#24812=CARTESIAN_POINT('',(7.93725393319377,0.,1.));
#24813=CARTESIAN_POINT('',(-7.93725393319377,0.,1.));
#24814=CARTESIAN_POINT('Origin',(0.,0.,0.));
#24815=CARTESIAN_POINT('',(0.,0.,1.));
#24816=CARTESIAN_POINT('Origin',(-10.8574973831368,0.,1.));
#24817=CARTESIAN_POINT('',(-7.93725393319377,2.,1.));
#24818=CARTESIAN_POINT('',(-10.8574973831368,2.,1.));
#24819=CARTESIAN_POINT('',(-10.8574973831368,30.,1.));
#24820=CARTESIAN_POINT('',(7.93725393319377,2.,1.));
#24821=CARTESIAN_POINT('',(-10.8574973831368,2.,1.));
#24822=CARTESIAN_POINT('',(7.93725393319377,2.,1.));
#24823=CARTESIAN_POINT('',(-7.93725393319377,2.,1.));
#24824=CARTESIAN_POINT('Origin',(0.,30.,0.));
#24825=CARTESIAN_POINT('Origin',(0.,2.,0.));
#24826=CARTESIAN_POINT('Origin',(0.,2.,0.));
#24827=CARTESIAN_POINT('Origin',(0.,2.,0.));
#24828=CARTESIAN_POINT('Origin',(0.,2.,0.));
#24829=CARTESIAN_POINT('',(-7.93725393319377,2.,-1.));
#24830=CARTESIAN_POINT('',(7.93725393319377,2.,-1.));
#24831=CARTESIAN_POINT('Origin',(0.,2.,0.));
#24832=CARTESIAN_POINT('',(7.93725393319377,0.,-1.));
#24833=CARTESIAN_POINT('',(7.93725393319377,2.,-1.));
#24834=CARTESIAN_POINT('',(-7.93725393319377,0.,-1.));
#24835=CARTESIAN_POINT('Origin',(0.,0.,0.));
#24836=CARTESIAN_POINT('',(-7.93725393319377,2.,-1.));
#24837=CARTESIAN_POINT('Origin',(0.,30.,0.));
#24838=CARTESIAN_POINT('',(9.94987437106619,30.,-1.));
#24839=CARTESIAN_POINT('',(-9.9498743710662,30.,-1.));
#24840=CARTESIAN_POINT('Origin',(0.,30.,0.));
#24841=CARTESIAN_POINT('',(9.9498743710662,2.,-1.));
#24842=CARTESIAN_POINT('',(9.9498743710662,30.,-1.));
#24843=CARTESIAN_POINT('',(-9.9498743710662,2.,-1.));
#24844=CARTESIAN_POINT('Origin',(0.,2.,0.));
#24845=CARTESIAN_POINT('',(-9.9498743710662,30.,-1.));
#24846=CARTESIAN_POINT('Origin',(0.,0.,0.));
#24847=CARTESIAN_POINT('',(0.,0.,-1.));
#24848=CARTESIAN_POINT('Origin',(-10.8574973831368,0.,-1.));
#24849=CARTESIAN_POINT('',(-10.8574973831368,2.,-1.));
#24850=CARTESIAN_POINT('',(-10.8574973831368,30.,-1.));
#24851=CARTESIAN_POINT('',(-10.8574973831368,2.,-1.));
#24852=CARTESIAN_POINT('Origin',(0.,30.,0.));
#24853=CARTESIAN_POINT('Origin',(0.,2.,0.));
#24854=CARTESIAN_POINT('Origin',(9.9498743710662,0.,1.));
#24855=CARTESIAN_POINT('',(9.9498743710662,2.,1.));
#24856=CARTESIAN_POINT('',(9.9498743710662,30.,1.));
#24857=CARTESIAN_POINT('',(9.9498743710662,0.,1.));
#24858=CARTESIAN_POINT('',(9.9498743710662,2.,-1.));
#24859=CARTESIAN_POINT('',(9.9498743710662,2.,1.));
#24860=CARTESIAN_POINT('',(9.9498743710662,30.,-1.));
#24861=CARTESIAN_POINT('',(9.9498743710662,0.,-1.));
#24862=CARTESIAN_POINT('',(9.9498743710662,30.,1.));
#24863=CARTESIAN_POINT('Origin',(-9.9498743710662,0.,1.));
#24864=CARTESIAN_POINT('',(-9.9498743710662,2.,1.));
#24865=CARTESIAN_POINT('',(-9.9498743710662,30.,1.));
#24866=CARTESIAN_POINT('',(-9.9498743710662,0.,1.));
#24867=CARTESIAN_POINT('',(-7.93725393319377,2.,1.));
#24868=CARTESIAN_POINT('',(-9.9498743710662,2.,1.));
#24869=CARTESIAN_POINT('',(-7.93725393319377,0.,1.));
#24870=CARTESIAN_POINT('',(-7.93725393319377,2.,1.));
#24871=CARTESIAN_POINT('',(7.93725393319377,0.,1.));
#24872=CARTESIAN_POINT('',(-9.9498743710662,0.,1.));
#24873=CARTESIAN_POINT('',(7.93725393319377,2.,1.));
#24874=CARTESIAN_POINT('',(7.93725393319377,2.,1.));
#24875=CARTESIAN_POINT('',(-9.9498743710662,2.,1.));
#24876=CARTESIAN_POINT('',(-9.9498743710662,30.,1.));
#24877=CARTESIAN_POINT('Origin',(-9.9498743710662,0.,1.));
#24878=CARTESIAN_POINT('',(-9.9498743710662,2.,-1.));
#24879=CARTESIAN_POINT('',(-9.9498743710662,30.,-1.));
#24880=CARTESIAN_POINT('',(-9.9498743710662,0.,-1.));
#24881=CARTESIAN_POINT('',(-9.9498743710662,2.,1.));
#24882=CARTESIAN_POINT('',(-9.9498743710662,30.,1.));
#24883=CARTESIAN_POINT('Origin',(-9.9498743710662,0.,-1.));
#24884=CARTESIAN_POINT('',(7.93725393319377,2.,-1.));
#24885=CARTESIAN_POINT('',(-9.9498743710662,2.,-1.));
#24886=CARTESIAN_POINT('',(7.93725393319377,0.,-1.));
#24887=CARTESIAN_POINT('',(7.93725393319377,2.,-1.));
#24888=CARTESIAN_POINT('',(-7.93725393319377,0.,-1.));
#24889=CARTESIAN_POINT('',(-9.9498743710662,0.,-1.));
#24890=CARTESIAN_POINT('',(-7.93725393319377,2.,-1.));
#24891=CARTESIAN_POINT('',(-7.93725393319377,2.,-1.));
#24892=CARTESIAN_POINT('',(-9.9498743710662,2.,-1.));
#24893=CARTESIAN_POINT('',(-9.9498743710662,30.,-1.));
#24894=CARTESIAN_POINT('Origin',(0.,0.,0.));
#24895=CARTESIAN_POINT('Origin',(0.,0.,0.));
#24896=CARTESIAN_POINT('Origin',(0.,0.,0.));
#24897=CARTESIAN_POINT('Origin',(0.,30.,0.));
#24898=CARTESIAN_POINT('Origin',(0.,2.,0.));
#24899=CARTESIAN_POINT('Origin',(0.,2.,0.));
#24900=CARTESIAN_POINT('Origin',(0.,2.,0.));
#24901=CARTESIAN_POINT('Origin',(0.,2.,0.));
#24902=CARTESIAN_POINT('Origin',(0.,2.,0.));
#24903=CARTESIAN_POINT('Origin',(0.,2.,0.));
#24904=CARTESIAN_POINT('Origin',(5.51672269044018,43.,2.35918858016532));
#24905=CARTESIAN_POINT('',(6.9531279684454,43.,2.97345743479371));
#24906=CARTESIAN_POINT('',(6.53903774184515,43.,-0.031391252358755));
#24907=CARTESIAN_POINT('',(6.53903774184515,43.,-0.0313912523587545));
#24908=CARTESIAN_POINT('Origin',(5.51672269044018,43.,2.35918858016532));
#24909=CARTESIAN_POINT('Origin',(-7.35563025392024,43.,-3.14558477355376));
#24910=CARTESIAN_POINT('',(-5.93400757601218,43.,-5.36540344129219));
#24911=CARTESIAN_POINT('',(-6.33331520251527,43.,-5.53616460607784));
#24912=CARTESIAN_POINT('Ctrl Pts',(-5.93400757601218,43.,-5.36540344129219));
#24913=CARTESIAN_POINT('Ctrl Pts',(-5.93400757601218,43.3291290637156,-5.36540344129219));
#24914=CARTESIAN_POINT('Ctrl Pts',(-5.98188388226438,43.6784012049209,-5.3138038536473));
#24915=CARTESIAN_POINT('Ctrl Pts',(-6.16344333601518,44.3181838212083,-5.10209873618755));
#24916=CARTESIAN_POINT('Ctrl Pts',(-6.29577793931752,44.6089260296629,-4.94153945058315));
#24917=CARTESIAN_POINT('Ctrl Pts',(-6.57591405287913,45.0679335530487,-4.56212012179661));
#24918=CARTESIAN_POINT('Ctrl Pts',(-6.74280768323277,45.2676678832806,-4.31723749028182));
#24919=CARTESIAN_POINT('Ctrl Pts',(-7.06842395635423,45.5337646559893,-3.76050232959795));
#24920=CARTESIAN_POINT('Ctrl Pts',(-7.22627127313154,45.6,-3.44807760118488));
#24921=CARTESIAN_POINT('Ctrl Pts',(-7.48498923470894,45.6,-2.84309194592264));
#24922=CARTESIAN_POINT('Ctrl Pts',(-7.60185005331357,45.5337646559893,-2.51313962298366));
#24923=CARTESIAN_POINT('Ctrl Pts',(-7.7794675367706,45.2676678832806,-1.89311379607514));
#24924=CARTESIAN_POINT('Ctrl Pts',(-7.84124260001151,45.0679335530487,-1.60327793108978));
#24925=CARTESIAN_POINT('Ctrl Pts',(-7.92206825557714,44.6089260296629,-1.13862485342795));
#24926=CARTESIAN_POINT('Ctrl Pts',(-7.94674595386654,44.3181838212083,-0.932026831578464));
#24927=CARTESIAN_POINT('Ctrl Pts',(-7.97440083953437,43.6784012049209,-0.654505482303069));
#24928=CARTESIAN_POINT('Ctrl Pts',(-7.97863767882213,43.3291290637156,-0.584243776244034));
#24929=CARTESIAN_POINT('Ctrl Pts',(-7.97863767882213,42.6708709362844,-0.584243776244034));
#24930=CARTESIAN_POINT('Ctrl Pts',(-7.97440083953437,42.3215987950791,-0.654505482303069));
#24931=CARTESIAN_POINT('Ctrl Pts',(-7.94674595386654,41.6818161787917,-0.932026831578464));
#24932=CARTESIAN_POINT('Ctrl Pts',(-7.92206825557714,41.3910739703371,-1.13862485342795));
#24933=CARTESIAN_POINT('Ctrl Pts',(-7.84124260001151,40.9320664469513,-1.60327793108978));
#24934=CARTESIAN_POINT('Ctrl Pts',(-7.7794675367706,40.7323321167194,-1.89311379607514));
#24935=CARTESIAN_POINT('Ctrl Pts',(-7.60185005331357,40.4662353440107,-2.51313962298366));
#24936=CARTESIAN_POINT('Ctrl Pts',(-7.48498923470894,40.4,-2.84309194592264));
#24937=CARTESIAN_POINT('Ctrl Pts',(-7.22627127313154,40.4,-3.44807760118488));
#24938=CARTESIAN_POINT('Ctrl Pts',(-7.06842395635423,40.4662353440107,-3.76050232959794));
#24939=CARTESIAN_POINT('Ctrl Pts',(-6.74280768323277,40.7323321167194,-4.31723749028181));
#24940=CARTESIAN_POINT('Ctrl Pts',(-6.57591405287913,40.9320664469513,-4.56212012179661));
#24941=CARTESIAN_POINT('Ctrl Pts',(-6.29577793931752,41.3910739703371,-4.94153945058315));
#24942=CARTESIAN_POINT('Ctrl Pts',(-6.16344333601518,41.6818161787917,-5.10209873618755));
#24943=CARTESIAN_POINT('Ctrl Pts',(-5.98188388226438,42.3215987950791,-5.3138038536473));
#24944=CARTESIAN_POINT('Ctrl Pts',(-5.93400757601218,42.6708709362844,-5.36540344129219));
#24945=CARTESIAN_POINT('Ctrl Pts',(-5.93400757601218,43.,-5.36540344129219));
#24946=CARTESIAN_POINT('Origin',(0.,48.,0.));
#24947=CARTESIAN_POINT('',(-9.79717439317883E-16,47.,8.));
#24948=CARTESIAN_POINT('Origin',(0.,47.,0.));
#24949=CARTESIAN_POINT('',(-8.57252759403147E-16,48.,7.));
#24950=CARTESIAN_POINT('',(-8.57252759403147E-16,48.,7.));
#24951=CARTESIAN_POINT('Origin',(0.,48.,0.));
#24952=CARTESIAN_POINT('Origin',(0.,32.,0.));
#24953=CARTESIAN_POINT('',(-1.20399315864541E-15,31.2588190451025,-9.66270045344786));
#24954=CARTESIAN_POINT('',(-1.18333951814346E-15,31.2588190451025,9.66270045344786));
#24955=CARTESIAN_POINT('Origin',(0.,31.2588190451025,0.));
#24956=CARTESIAN_POINT('Origin',(0.,31.2588190451025,0.));
#24957=CARTESIAN_POINT('',(-1.06504772100559E-15,32.,8.69677462715879));
#24958=CARTESIAN_POINT('',(-1.06504772100559E-15,32.,8.69677462715879));
#24959=CARTESIAN_POINT('Origin',(0.,32.,0.));
#24960=CARTESIAN_POINT('Origin',(0.,48.,0.));
#24961=CARTESIAN_POINT('',(-9.79717439317883E-16,32.,8.));
#24962=CARTESIAN_POINT('Origin',(0.,32.,0.));
#24963=CARTESIAN_POINT('',(-9.79717439317883E-16,48.,8.));
#24964=CARTESIAN_POINT('Origin',(0.,30.,0.));
#24965=CARTESIAN_POINT('',(1.22464679914735E-15,30.,-10.));
#24966=CARTESIAN_POINT('Origin',(0.,30.,0.));
#24967=CARTESIAN_POINT('',(1.22464679914735E-15,30.,-10.));
#24968=CARTESIAN_POINT('Origin',(0.,32.,0.));
#24969=CARTESIAN_POINT('Origin',(0.,30.,0.));
#24970=CARTESIAN_POINT('Origin',(0.,48.,0.));
#38606=UNCERTAINTY_MEASURE_WITH_UNIT(LENGTH_MEASURE(0.01),#38636,
'DISTANCE_ACCURACY_VALUE',
'Maximum model space distance between geometric entities at asserted c
onnectivities');
#38619=UNCERTAINTY_MEASURE_WITH_UNIT(LENGTH_MEASURE(0.01),#38636,
'DISTANCE_ACCURACY_VALUE',
'Maximum model space distance between geometric entities at asserted c
onnectivities');
#38622=(
GEOMETRIC_REPRESENTATION_CONTEXT(3)
GLOBAL_UNCERTAINTY_ASSIGNED_CONTEXT((#38606))
GLOBAL_UNIT_ASSIGNED_CONTEXT((#38636,#38638,#38639))
REPRESENTATION_CONTEXT('','3D')
);
#38635=(
GEOMETRIC_REPRESENTATION_CONTEXT(3)
GLOBAL_UNCERTAINTY_ASSIGNED_CONTEXT((#38619))
GLOBAL_UNIT_ASSIGNED_CONTEXT((#38636,#38638,#38639))
REPRESENTATION_CONTEXT('','3D')
);
#38636=(
LENGTH_UNIT()
NAMED_UNIT(*)
SI_UNIT(.MILLI.,.METRE.)
);
#38638=(
NAMED_UNIT(*)
PLANE_ANGLE_UNIT()
SI_UNIT($,.RADIAN.)
);
#38639=(
NAMED_UNIT(*)
SI_UNIT($,.STERADIAN.)
SOLID_ANGLE_UNIT()
);
#38642=SHAPE_DEFINITION_REPRESENTATION(#38657,#38686);
#38657=PRODUCT_DEFINITION_SHAPE('',$,#38702);
#38686=SHAPE_REPRESENTATION('',(#17857),#38622);
#38699=PRODUCT_DEFINITION_CONTEXT('part definition',#38746,'design');
#38702=PRODUCT_DEFINITION('Magnetic Base Core','Magnetic Base Core',#38717,
#38699);
#38717=PRODUCT_DEFINITION_FORMATION('',$,#38750);
#38746=APPLICATION_CONTEXT(
'Core Data for Automotive Mechanical Design Process');
#38747=PRODUCT_CONTEXT('part definition',#38746,'mechanical');
#38750=PRODUCT('Magnetic Base Core','Magnetic Base Core',$,(#38747));
#38765=PRESENTATION_STYLE_ASSIGNMENT((#38772));
#38772=SURFACE_STYLE_USAGE(.BOTH.,#38779);
#38779=SURFACE_SIDE_STYLE('',(#38786));
#38786=SURFACE_STYLE_FILL_AREA(#38793);
#38793=FILL_AREA_STYLE('Opaque(227,224,212)',(#38800));
#38800=FILL_AREA_STYLE_COLOUR('Opaque(227,224,212)',#38807);
#38807=COLOUR_RGB('Opaque(227,224,212)',0.890196078431372,0.87843137254902,
0.831372549019608);
ENDSEC;
END-ISO-10303-21;
